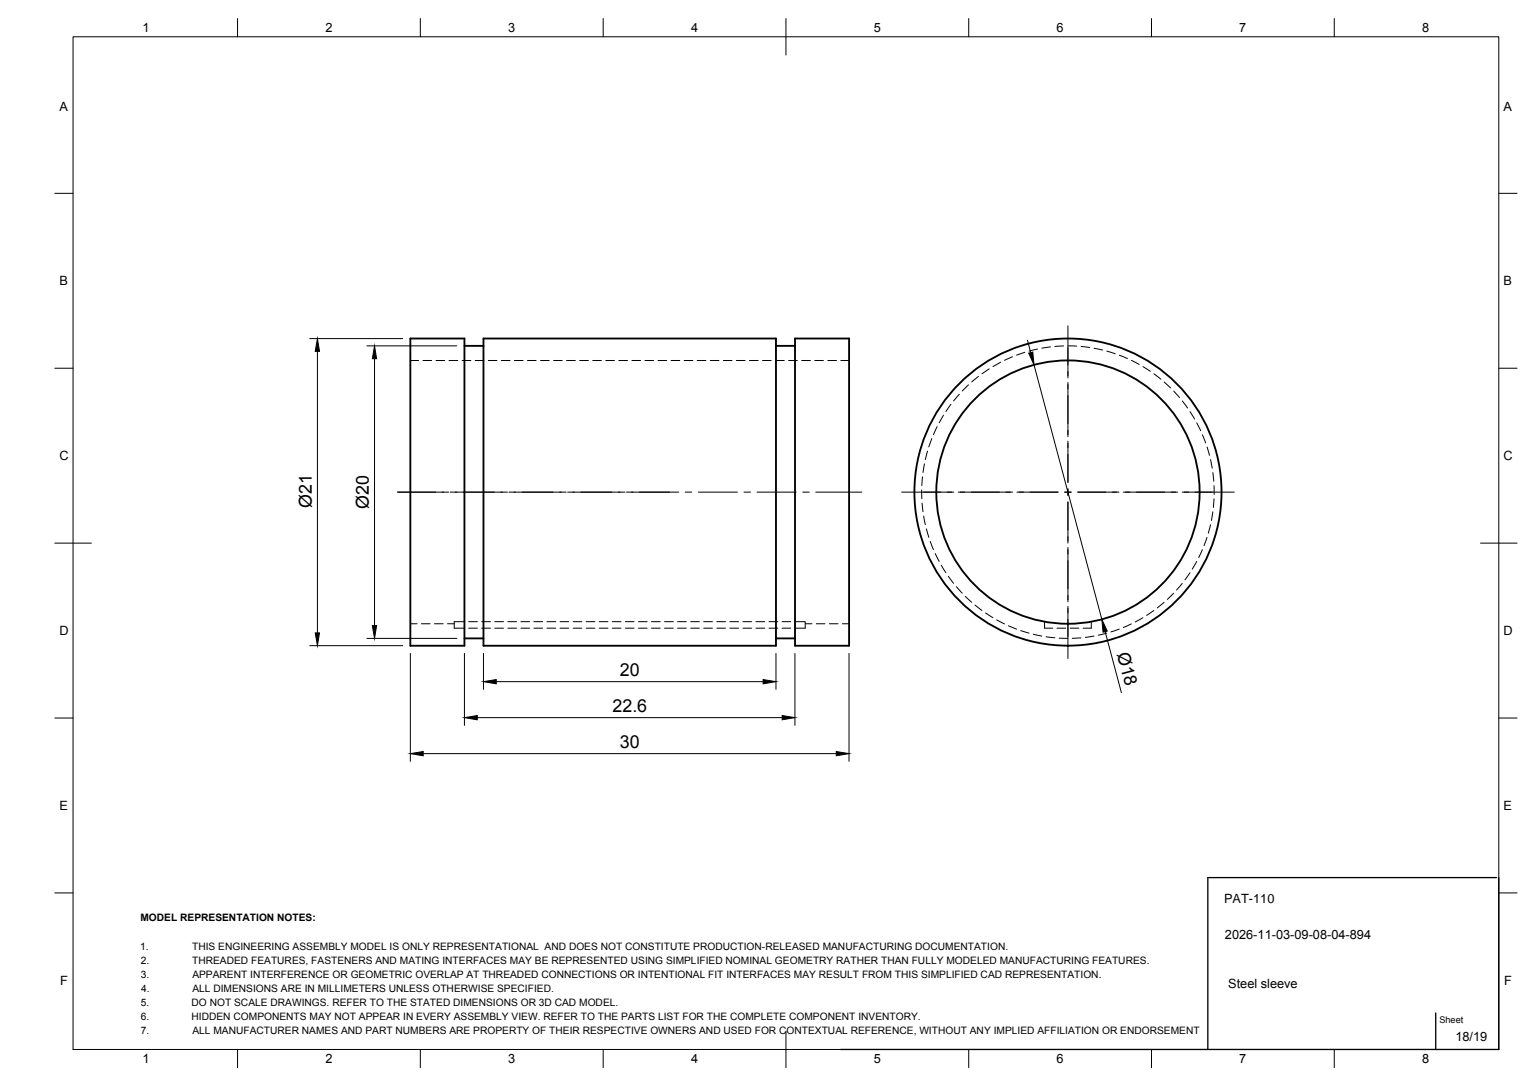
ISO-10303-21;
HEADER;
/* Generated by software containing ST-Developer
 * from STEP Tools, Inc. (www.steptools.com) 
 */

FILE_DESCRIPTION(
/* description */ ('Twin-shaft manual slide'),
/* implementation_level */ '2;1');

FILE_NAME(
/* name */ 'Steel sleeve.step',
/* time_stamp */ '2026-10-27T18:38:08-07:00',
/* author */ (''),
/* organization */ (''),
/* preprocessor_version */ 'ST-DEVELOPER v20.2',
/* originating_system */ 'Autodesk Translation Framework v15.17.0.0',
/* authorisation */ '');

FILE_SCHEMA (('AUTOMOTIVE_DESIGN { 1 0 10303 214 3 1 1 }'));
ENDSEC;

DATA;
#10=MECHANICAL_DESIGN_GEOMETRIC_PRESENTATION_REPRESENTATION('',(#284),#6463);
#252=SHAPE_REPRESENTATION_RELATIONSHIP('SRR','None',#6572,#268);
#268=ADVANCED_BREP_SHAPE_REPRESENTATION('',(#299),#6455);
#284=STYLED_ITEM('',(#6754),#299);
#299=MANIFOLD_SOLID_BREP('Body1',#3647);
#371=FACE_BOUND('',#917,.T.);
#372=FACE_BOUND('',#920,.T.);
#373=FACE_BOUND('',#923,.T.);
#374=FACE_BOUND('',#926,.T.);
#375=FACE_BOUND('',#929,.T.);
#376=FACE_BOUND('',#932,.T.);
#377=FACE_BOUND('',#934,.T.);
#466=PLANE('',#4046);
#467=PLANE('',#4048);
#468=PLANE('',#4049);
#469=PLANE('',#4051);
#470=PLANE('',#4052);
#471=PLANE('',#4053);
#472=PLANE('',#4058);
#473=PLANE('',#4062);
#474=PLANE('',#4066);
#475=PLANE('',#4070);
#476=PLANE('',#4074);
#637=FACE_OUTER_BOUND('',#911,.T.);
#638=FACE_OUTER_BOUND('',#912,.T.);
#639=FACE_OUTER_BOUND('',#913,.T.);
#640=FACE_OUTER_BOUND('',#914,.T.);
#641=FACE_OUTER_BOUND('',#915,.T.);
#642=FACE_OUTER_BOUND('',#916,.T.);
#643=FACE_OUTER_BOUND('',#918,.T.);
#644=FACE_OUTER_BOUND('',#919,.T.);
#645=FACE_OUTER_BOUND('',#921,.T.);
#646=FACE_OUTER_BOUND('',#922,.T.);
#647=FACE_OUTER_BOUND('',#924,.T.);
#648=FACE_OUTER_BOUND('',#925,.T.);
#649=FACE_OUTER_BOUND('',#927,.T.);
#650=FACE_OUTER_BOUND('',#928,.T.);
#651=FACE_OUTER_BOUND('',#930,.T.);
#652=FACE_OUTER_BOUND('',#931,.T.);
#653=FACE_OUTER_BOUND('',#933,.T.);
#911=EDGE_LOOP('',(#2994,#2995,#2996,#2997));
#912=EDGE_LOOP('',(#2998,#2999,#3000,#3001));
#913=EDGE_LOOP('',(#3002,#3003,#3004,#3005));
#914=EDGE_LOOP('',(#3006,#3007,#3008,#3009));
#915=EDGE_LOOP('',(#3010,#3011,#3012,#3013));
#916=EDGE_LOOP('',(#3014));
#917=EDGE_LOOP('',(#3015));
#918=EDGE_LOOP('',(#3016,#3017,#3018,#3019));
#919=EDGE_LOOP('',(#3020));
#920=EDGE_LOOP('',(#3021));
#921=EDGE_LOOP('',(#3022,#3023,#3024,#3025));
#922=EDGE_LOOP('',(#3026));
#923=EDGE_LOOP('',(#3027));
#924=EDGE_LOOP('',(#3028,#3029,#3030,#3031));
#925=EDGE_LOOP('',(#3032));
#926=EDGE_LOOP('',(#3033));
#927=EDGE_LOOP('',(#3034,#3035,#3036,#3037));
#928=EDGE_LOOP('',(#3038));
#929=EDGE_LOOP('',(#3039));
#930=EDGE_LOOP('',(#3040,#3041,#3042,#3043));
#931=EDGE_LOOP('',(#3044));
#932=EDGE_LOOP('',(#3045));
#933=EDGE_LOOP('',(#3046,#3047,#3048,#3049));
#934=EDGE_LOOP('',(#3050,#3051,#3052,#3053));
#1203=LINE('',#5966,#1489);
#1204=LINE('',#5968,#1490);
#1205=LINE('',#5969,#1491);
#1206=LINE('',#5972,#1492);
#1207=LINE('',#5974,#1493);
#1208=LINE('',#5975,#1494);
#1209=LINE('',#5980,#1495);
#1210=LINE('',#5981,#1496);
#1211=LINE('',#5983,#1497);
#1212=LINE('',#5984,#1498);
#1213=LINE('',#5994,#1499);
#1214=LINE('',#6001,#1500);
#1215=LINE('',#6008,#1501);
#1216=LINE('',#6015,#1502);
#1217=LINE('',#6022,#1503);
#1218=LINE('',#6027,#1504);
#1489=VECTOR('',#4859,1.);
#1490=VECTOR('',#4860,1.);
#1491=VECTOR('',#4861,1.);
#1492=VECTOR('',#4864,1.);
#1493=VECTOR('',#4865,1.);
#1494=VECTOR('',#4866,1.);
#1495=VECTOR('',#4871,1.);
#1496=VECTOR('',#4872,1.);
#1497=VECTOR('',#4875,1.);
#1498=VECTOR('',#4876,1.);
#1499=VECTOR('',#4889,1.05);
#1500=VECTOR('',#4898,1.);
#1501=VECTOR('',#4907,1.05);
#1502=VECTOR('',#4916,1.);
#1503=VECTOR('',#4925,1.05);
#1504=VECTOR('',#4932,0.9);
#1696=CIRCLE('',#4047,0.9);
#1697=CIRCLE('',#4050,0.9);
#1698=CIRCLE('',#4054,1.05);
#1699=CIRCLE('',#4055,0.9);
#1700=CIRCLE('',#4057,1.05);
#1701=CIRCLE('',#4059,1.);
#1702=CIRCLE('',#4061,1.);
#1703=CIRCLE('',#4063,1.05);
#1704=CIRCLE('',#4065,1.05);
#1705=CIRCLE('',#4067,1.);
#1706=CIRCLE('',#4069,1.);
#1707=CIRCLE('',#4071,1.05);
#1708=CIRCLE('',#4073,1.05);
#1709=CIRCLE('',#4075,0.9);
#1929=VERTEX_POINT('',#5962);
#1930=VERTEX_POINT('',#5963);
#1931=VERTEX_POINT('',#5965);
#1932=VERTEX_POINT('',#5967);
#1933=VERTEX_POINT('',#5971);
#1934=VERTEX_POINT('',#5973);
#1935=VERTEX_POINT('',#5977);
#1936=VERTEX_POINT('',#5979);
#1937=VERTEX_POINT('',#5987);
#1938=VERTEX_POINT('',#5989);
#1939=VERTEX_POINT('',#5992);
#1940=VERTEX_POINT('',#5996);
#1941=VERTEX_POINT('',#5999);
#1942=VERTEX_POINT('',#6003);
#1943=VERTEX_POINT('',#6006);
#1944=VERTEX_POINT('',#6010);
#1945=VERTEX_POINT('',#6013);
#1946=VERTEX_POINT('',#6017);
#1947=VERTEX_POINT('',#6020);
#1948=VERTEX_POINT('',#6024);
#2302=EDGE_CURVE('',#1929,#1930,#1696,.T.);
#2303=EDGE_CURVE('',#1931,#1929,#1203,.T.);
#2304=EDGE_CURVE('',#1932,#1931,#1204,.T.);
#2305=EDGE_CURVE('',#1930,#1932,#1205,.T.);
#2306=EDGE_CURVE('',#1930,#1933,#1206,.T.);
#2307=EDGE_CURVE('',#1934,#1932,#1207,.T.);
#2308=EDGE_CURVE('',#1934,#1933,#1208,.T.);
#2309=EDGE_CURVE('',#1933,#1935,#1697,.T.);
#2310=EDGE_CURVE('',#1936,#1934,#1209,.T.);
#2311=EDGE_CURVE('',#1935,#1936,#1210,.T.);
#2312=EDGE_CURVE('',#1935,#1929,#1211,.T.);
#2313=EDGE_CURVE('',#1936,#1931,#1212,.T.);
#2314=EDGE_CURVE('',#1937,#1937,#1698,.T.);
#2315=EDGE_CURVE('',#1938,#1938,#1699,.T.);
#2316=EDGE_CURVE('',#1939,#1939,#1700,.T.);
#2317=EDGE_CURVE('',#1939,#1937,#1213,.T.);
#2318=EDGE_CURVE('',#1940,#1940,#1701,.T.);
#2319=EDGE_CURVE('',#1941,#1941,#1702,.T.);
#2320=EDGE_CURVE('',#1941,#1940,#1214,.T.);
#2321=EDGE_CURVE('',#1942,#1942,#1703,.T.);
#2322=EDGE_CURVE('',#1943,#1943,#1704,.T.);
#2323=EDGE_CURVE('',#1943,#1942,#1215,.T.);
#2324=EDGE_CURVE('',#1944,#1944,#1705,.T.);
#2325=EDGE_CURVE('',#1945,#1945,#1706,.T.);
#2326=EDGE_CURVE('',#1945,#1944,#1216,.T.);
#2327=EDGE_CURVE('',#1946,#1946,#1707,.T.);
#2328=EDGE_CURVE('',#1947,#1947,#1708,.T.);
#2329=EDGE_CURVE('',#1947,#1946,#1217,.T.);
#2330=EDGE_CURVE('',#1948,#1948,#1709,.T.);
#2331=EDGE_CURVE('',#1948,#1938,#1218,.T.);
#2994=ORIENTED_EDGE('',*,*,#2302,.F.);
#2995=ORIENTED_EDGE('',*,*,#2303,.F.);
#2996=ORIENTED_EDGE('',*,*,#2304,.F.);
#2997=ORIENTED_EDGE('',*,*,#2305,.F.);
#2998=ORIENTED_EDGE('',*,*,#2306,.F.);
#2999=ORIENTED_EDGE('',*,*,#2305,.T.);
#3000=ORIENTED_EDGE('',*,*,#2307,.F.);
#3001=ORIENTED_EDGE('',*,*,#2308,.T.);
#3002=ORIENTED_EDGE('',*,*,#2309,.F.);
#3003=ORIENTED_EDGE('',*,*,#2308,.F.);
#3004=ORIENTED_EDGE('',*,*,#2310,.F.);
#3005=ORIENTED_EDGE('',*,*,#2311,.F.);
#3006=ORIENTED_EDGE('',*,*,#2312,.F.);
#3007=ORIENTED_EDGE('',*,*,#2311,.T.);
#3008=ORIENTED_EDGE('',*,*,#2313,.T.);
#3009=ORIENTED_EDGE('',*,*,#2303,.T.);
#3010=ORIENTED_EDGE('',*,*,#2313,.F.);
#3011=ORIENTED_EDGE('',*,*,#2310,.T.);
#3012=ORIENTED_EDGE('',*,*,#2307,.T.);
#3013=ORIENTED_EDGE('',*,*,#2304,.T.);
#3014=ORIENTED_EDGE('',*,*,#2314,.F.);
#3015=ORIENTED_EDGE('',*,*,#2315,.T.);
#3016=ORIENTED_EDGE('',*,*,#2316,.F.);
#3017=ORIENTED_EDGE('',*,*,#2317,.T.);
#3018=ORIENTED_EDGE('',*,*,#2314,.T.);
#3019=ORIENTED_EDGE('',*,*,#2317,.F.);
#3020=ORIENTED_EDGE('',*,*,#2316,.T.);
#3021=ORIENTED_EDGE('',*,*,#2318,.F.);
#3022=ORIENTED_EDGE('',*,*,#2319,.F.);
#3023=ORIENTED_EDGE('',*,*,#2320,.T.);
#3024=ORIENTED_EDGE('',*,*,#2318,.T.);
#3025=ORIENTED_EDGE('',*,*,#2320,.F.);
#3026=ORIENTED_EDGE('',*,*,#2321,.F.);
#3027=ORIENTED_EDGE('',*,*,#2319,.T.);
#3028=ORIENTED_EDGE('',*,*,#2322,.F.);
#3029=ORIENTED_EDGE('',*,*,#2323,.T.);
#3030=ORIENTED_EDGE('',*,*,#2321,.T.);
#3031=ORIENTED_EDGE('',*,*,#2323,.F.);
#3032=ORIENTED_EDGE('',*,*,#2322,.T.);
#3033=ORIENTED_EDGE('',*,*,#2324,.F.);
#3034=ORIENTED_EDGE('',*,*,#2325,.F.);
#3035=ORIENTED_EDGE('',*,*,#2326,.T.);
#3036=ORIENTED_EDGE('',*,*,#2324,.T.);
#3037=ORIENTED_EDGE('',*,*,#2326,.F.);
#3038=ORIENTED_EDGE('',*,*,#2327,.F.);
#3039=ORIENTED_EDGE('',*,*,#2325,.T.);
#3040=ORIENTED_EDGE('',*,*,#2328,.F.);
#3041=ORIENTED_EDGE('',*,*,#2329,.T.);
#3042=ORIENTED_EDGE('',*,*,#2327,.T.);
#3043=ORIENTED_EDGE('',*,*,#2329,.F.);
#3044=ORIENTED_EDGE('',*,*,#2328,.T.);
#3045=ORIENTED_EDGE('',*,*,#2330,.F.);
#3046=ORIENTED_EDGE('',*,*,#2330,.T.);
#3047=ORIENTED_EDGE('',*,*,#2331,.T.);
#3048=ORIENTED_EDGE('',*,*,#2315,.F.);
#3049=ORIENTED_EDGE('',*,*,#2331,.F.);
#3050=ORIENTED_EDGE('',*,*,#2309,.T.);
#3051=ORIENTED_EDGE('',*,*,#2312,.T.);
#3052=ORIENTED_EDGE('',*,*,#2302,.T.);
#3053=ORIENTED_EDGE('',*,*,#2306,.T.);
#3407=CYLINDRICAL_SURFACE('',#4056,1.05);
#3408=CYLINDRICAL_SURFACE('',#4060,1.);
#3409=CYLINDRICAL_SURFACE('',#4064,1.05);
#3410=CYLINDRICAL_SURFACE('',#4068,1.);
#3411=CYLINDRICAL_SURFACE('',#4072,1.05);
#3412=CYLINDRICAL_SURFACE('',#4076,0.9);
#3542=ADVANCED_FACE('',(#637),#466,.F.);
#3543=ADVANCED_FACE('',(#638),#467,.F.);
#3544=ADVANCED_FACE('',(#639),#468,.F.);
#3545=ADVANCED_FACE('',(#640),#469,.F.);
#3546=ADVANCED_FACE('',(#641),#470,.F.);
#3547=ADVANCED_FACE('',(#642,#371),#471,.T.);
#3548=ADVANCED_FACE('',(#643),#3407,.T.);
#3549=ADVANCED_FACE('',(#644,#372),#472,.T.);
#3550=ADVANCED_FACE('',(#645),#3408,.T.);
#3551=ADVANCED_FACE('',(#646,#373),#473,.T.);
#3552=ADVANCED_FACE('',(#647),#3409,.T.);
#3553=ADVANCED_FACE('',(#648,#374),#474,.T.);
#3554=ADVANCED_FACE('',(#649),#3410,.T.);
#3555=ADVANCED_FACE('',(#650,#375),#475,.T.);
#3556=ADVANCED_FACE('',(#651),#3411,.T.);
#3557=ADVANCED_FACE('',(#652,#376),#476,.T.);
#3558=ADVANCED_FACE('',(#653,#377),#3412,.F.);
#3647=CLOSED_SHELL('',(#3542,#3543,#3544,#3545,#3546,#3547,#3548,#3549,
#3550,#3551,#3552,#3553,#3554,#3555,#3556,#3557,#3558));
#4045=AXIS2_PLACEMENT_3D('',#5960,#4853,#4854);
#4046=AXIS2_PLACEMENT_3D('',#5961,#4855,#4856);
#4047=AXIS2_PLACEMENT_3D('',#5964,#4857,#4858);
#4048=AXIS2_PLACEMENT_3D('',#5970,#4862,#4863);
#4049=AXIS2_PLACEMENT_3D('',#5976,#4867,#4868);
#4050=AXIS2_PLACEMENT_3D('',#5978,#4869,#4870);
#4051=AXIS2_PLACEMENT_3D('',#5982,#4873,#4874);
#4052=AXIS2_PLACEMENT_3D('',#5985,#4877,#4878);
#4053=AXIS2_PLACEMENT_3D('',#5986,#4879,#4880);
#4054=AXIS2_PLACEMENT_3D('',#5988,#4881,#4882);
#4055=AXIS2_PLACEMENT_3D('',#5990,#4883,#4884);
#4056=AXIS2_PLACEMENT_3D('',#5991,#4885,#4886);
#4057=AXIS2_PLACEMENT_3D('',#5993,#4887,#4888);
#4058=AXIS2_PLACEMENT_3D('',#5995,#4890,#4891);
#4059=AXIS2_PLACEMENT_3D('',#5997,#4892,#4893);
#4060=AXIS2_PLACEMENT_3D('',#5998,#4894,#4895);
#4061=AXIS2_PLACEMENT_3D('',#6000,#4896,#4897);
#4062=AXIS2_PLACEMENT_3D('',#6002,#4899,#4900);
#4063=AXIS2_PLACEMENT_3D('',#6004,#4901,#4902);
#4064=AXIS2_PLACEMENT_3D('',#6005,#4903,#4904);
#4065=AXIS2_PLACEMENT_3D('',#6007,#4905,#4906);
#4066=AXIS2_PLACEMENT_3D('',#6009,#4908,#4909);
#4067=AXIS2_PLACEMENT_3D('',#6011,#4910,#4911);
#4068=AXIS2_PLACEMENT_3D('',#6012,#4912,#4913);
#4069=AXIS2_PLACEMENT_3D('',#6014,#4914,#4915);
#4070=AXIS2_PLACEMENT_3D('',#6016,#4917,#4918);
#4071=AXIS2_PLACEMENT_3D('',#6018,#4919,#4920);
#4072=AXIS2_PLACEMENT_3D('',#6019,#4921,#4922);
#4073=AXIS2_PLACEMENT_3D('',#6021,#4923,#4924);
#4074=AXIS2_PLACEMENT_3D('',#6023,#4926,#4927);
#4075=AXIS2_PLACEMENT_3D('',#6025,#4928,#4929);
#4076=AXIS2_PLACEMENT_3D('',#6026,#4930,#4931);
#4853=DIRECTION('axis',(0.,0.,1.));
#4854=DIRECTION('refdir',(1.,0.,0.));
#4855=DIRECTION('center_axis',(0.,1.,0.));
#4856=DIRECTION('ref_axis',(0.,0.,1.));
#4857=DIRECTION('center_axis',(0.,-1.,0.));
#4858=DIRECTION('ref_axis',(1.,0.,0.));
#4859=DIRECTION('',(-1.,0.,0.));
#4860=DIRECTION('',(0.,0.,-1.));
#4861=DIRECTION('',(1.,0.,0.));
#4862=DIRECTION('center_axis',(0.,0.,1.));
#4863=DIRECTION('ref_axis',(1.,0.,0.));
#4864=DIRECTION('',(0.,-1.,0.));
#4865=DIRECTION('',(0.,1.,0.));
#4866=DIRECTION('',(-1.,0.,0.));
#4867=DIRECTION('center_axis',(0.,-1.,0.));
#4868=DIRECTION('ref_axis',(0.,0.,-1.));
#4869=DIRECTION('center_axis',(0.,1.,0.));
#4870=DIRECTION('ref_axis',(1.,0.,0.));
#4871=DIRECTION('',(0.,0.,1.));
#4872=DIRECTION('',(1.,0.,0.));
#4873=DIRECTION('center_axis',(0.,0.,-1.));
#4874=DIRECTION('ref_axis',(-1.,0.,0.));
#4875=DIRECTION('',(0.,1.,0.));
#4876=DIRECTION('',(0.,1.,0.));
#4877=DIRECTION('center_axis',(1.,0.,0.));
#4878=DIRECTION('ref_axis',(0.,0.,-1.));
#4879=DIRECTION('center_axis',(0.,1.,0.));
#4880=DIRECTION('ref_axis',(0.,0.,1.));
#4881=DIRECTION('center_axis',(0.,-1.,0.));
#4882=DIRECTION('ref_axis',(1.,0.,0.));
#4883=DIRECTION('center_axis',(0.,-1.,0.));
#4884=DIRECTION('ref_axis',(1.,0.,0.));
#4885=DIRECTION('center_axis',(0.,-1.,0.));
#4886=DIRECTION('ref_axis',(1.,0.,0.));
#4887=DIRECTION('center_axis',(0.,-1.,0.));
#4888=DIRECTION('ref_axis',(1.,0.,0.));
#4889=DIRECTION('',(0.,1.,0.));
#4890=DIRECTION('center_axis',(0.,-1.,0.));
#4891=DIRECTION('ref_axis',(0.,0.,-1.));
#4892=DIRECTION('center_axis',(0.,-1.,0.));
#4893=DIRECTION('ref_axis',(1.,0.,0.));
#4894=DIRECTION('center_axis',(0.,-1.,0.));
#4895=DIRECTION('ref_axis',(1.,0.,0.));
#4896=DIRECTION('center_axis',(0.,-1.,0.));
#4897=DIRECTION('ref_axis',(1.,0.,0.));
#4898=DIRECTION('',(0.,1.,0.));
#4899=DIRECTION('center_axis',(0.,1.,0.));
#4900=DIRECTION('ref_axis',(0.,0.,1.));
#4901=DIRECTION('center_axis',(0.,-1.,0.));
#4902=DIRECTION('ref_axis',(1.,0.,0.));
#4903=DIRECTION('center_axis',(0.,-1.,0.));
#4904=DIRECTION('ref_axis',(1.,0.,0.));
#4905=DIRECTION('center_axis',(0.,-1.,0.));
#4906=DIRECTION('ref_axis',(1.,0.,0.));
#4907=DIRECTION('',(0.,1.,0.));
#4908=DIRECTION('center_axis',(0.,-1.,0.));
#4909=DIRECTION('ref_axis',(0.,0.,-1.));
#4910=DIRECTION('center_axis',(0.,-1.,0.));
#4911=DIRECTION('ref_axis',(1.,0.,0.));
#4912=DIRECTION('center_axis',(0.,-1.,0.));
#4913=DIRECTION('ref_axis',(1.,0.,0.));
#4914=DIRECTION('center_axis',(0.,-1.,0.));
#4915=DIRECTION('ref_axis',(1.,0.,0.));
#4916=DIRECTION('',(0.,1.,0.));
#4917=DIRECTION('center_axis',(0.,1.,0.));
#4918=DIRECTION('ref_axis',(0.,0.,1.));
#4919=DIRECTION('center_axis',(0.,-1.,0.));
#4920=DIRECTION('ref_axis',(1.,0.,0.));
#4921=DIRECTION('center_axis',(0.,-1.,0.));
#4922=DIRECTION('ref_axis',(1.,0.,0.));
#4923=DIRECTION('center_axis',(0.,-1.,0.));
#4924=DIRECTION('ref_axis',(1.,0.,0.));
#4925=DIRECTION('',(0.,1.,0.));
#4926=DIRECTION('center_axis',(0.,-1.,0.));
#4927=DIRECTION('ref_axis',(0.,0.,-1.));
#4928=DIRECTION('center_axis',(0.,-1.,0.));
#4929=DIRECTION('ref_axis',(1.,0.,0.));
#4930=DIRECTION('center_axis',(0.,-1.,0.));
#4931=DIRECTION('ref_axis',(1.,0.,0.));
#4932=DIRECTION('',(0.,1.,0.));
#5960=CARTESIAN_POINT('',(0.,0.,0.));
#5961=CARTESIAN_POINT('Origin',(0.75,1.2,0.));
#5962=CARTESIAN_POINT('',(0.885663593019381,1.2,-0.16));
#5963=CARTESIAN_POINT('',(0.885663593019381,1.2,0.16));
#5964=CARTESIAN_POINT('Origin',(0.,1.2,0.));
#5965=CARTESIAN_POINT('',(0.93,1.2,-0.16));
#5966=CARTESIAN_POINT('',(0.93,1.2,-0.16));
#5967=CARTESIAN_POINT('',(0.93,1.2,0.16));
#5968=CARTESIAN_POINT('',(0.93,1.2,0.16));
#5969=CARTESIAN_POINT('',(0.57,1.2,0.16));
#5970=CARTESIAN_POINT('Origin',(0.57,0.,0.16));
#5971=CARTESIAN_POINT('',(0.885663593019381,-1.2,0.16));
#5972=CARTESIAN_POINT('',(0.885663593019381,0.,0.16));
#5973=CARTESIAN_POINT('',(0.93,-1.2,0.16));
#5974=CARTESIAN_POINT('',(0.93,0.,0.16));
#5975=CARTESIAN_POINT('',(0.57,-1.2,0.16));
#5976=CARTESIAN_POINT('Origin',(0.75,-1.2,0.));
#5977=CARTESIAN_POINT('',(0.885663593019381,-1.2,-0.16));
#5978=CARTESIAN_POINT('Origin',(0.,-1.2,0.));
#5979=CARTESIAN_POINT('',(0.93,-1.2,-0.16));
#5980=CARTESIAN_POINT('',(0.93,-1.2,0.16));
#5981=CARTESIAN_POINT('',(0.93,-1.2,-0.16));
#5982=CARTESIAN_POINT('Origin',(0.93,0.,-0.16));
#5983=CARTESIAN_POINT('',(0.885663593019381,0.,-0.16));
#5984=CARTESIAN_POINT('',(0.93,0.,-0.16));
#5985=CARTESIAN_POINT('Origin',(0.93,0.,0.16));
#5986=CARTESIAN_POINT('Origin',(1.05,1.5,0.));
#5987=CARTESIAN_POINT('',(-1.05,1.5,-1.28587913910472E-16));
#5988=CARTESIAN_POINT('Origin',(0.,1.5,0.));
#5989=CARTESIAN_POINT('',(-0.9,1.5,-1.10218211923262E-16));
#5990=CARTESIAN_POINT('Origin',(0.,1.5,0.));
#5991=CARTESIAN_POINT('Origin',(0.,1.315,0.));
#5992=CARTESIAN_POINT('',(-1.05,1.13,-1.28587913910472E-16));
#5993=CARTESIAN_POINT('Origin',(0.,1.13,0.));
#5994=CARTESIAN_POINT('',(-1.05,1.315,-1.28587913910472E-16));
#5995=CARTESIAN_POINT('Origin',(1.,1.13,0.));
#5996=CARTESIAN_POINT('',(-1.,1.13,-1.22464679914735E-16));
#5997=CARTESIAN_POINT('Origin',(0.,1.13,0.));
#5998=CARTESIAN_POINT('Origin',(0.,1.065,0.));
#5999=CARTESIAN_POINT('',(-1.,1.,-1.22464679914735E-16));
#6000=CARTESIAN_POINT('Origin',(0.,1.,0.));
#6001=CARTESIAN_POINT('',(-1.,1.065,-1.22464679914735E-16));
#6002=CARTESIAN_POINT('Origin',(1.05,1.,0.));
#6003=CARTESIAN_POINT('',(-1.05,1.,-1.28587913910472E-16));
#6004=CARTESIAN_POINT('Origin',(0.,1.,0.));
#6005=CARTESIAN_POINT('Origin',(0.,0.,0.));
#6006=CARTESIAN_POINT('',(-1.05,-1.,-1.28587913910472E-16));
#6007=CARTESIAN_POINT('Origin',(0.,-1.,0.));
#6008=CARTESIAN_POINT('',(-1.05,0.,-1.28587913910472E-16));
#6009=CARTESIAN_POINT('Origin',(1.,-1.,0.));
#6010=CARTESIAN_POINT('',(-1.,-1.,-1.22464679914735E-16));
#6011=CARTESIAN_POINT('Origin',(0.,-1.,0.));
#6012=CARTESIAN_POINT('Origin',(0.,-1.065,0.));
#6013=CARTESIAN_POINT('',(-1.,-1.13,-1.22464679914735E-16));
#6014=CARTESIAN_POINT('Origin',(0.,-1.13,0.));
#6015=CARTESIAN_POINT('',(-1.,-1.065,-1.22464679914735E-16));
#6016=CARTESIAN_POINT('Origin',(1.05,-1.13,0.));
#6017=CARTESIAN_POINT('',(-1.05,-1.13,-1.28587913910472E-16));
#6018=CARTESIAN_POINT('Origin',(0.,-1.13,0.));
#6019=CARTESIAN_POINT('Origin',(0.,-1.315,0.));
#6020=CARTESIAN_POINT('',(-1.05,-1.5,-1.28587913910472E-16));
#6021=CARTESIAN_POINT('Origin',(0.,-1.5,0.));
#6022=CARTESIAN_POINT('',(-1.05,-1.315,-1.28587913910472E-16));
#6023=CARTESIAN_POINT('Origin',(0.9,-1.5,0.));
#6024=CARTESIAN_POINT('',(-0.9,-1.5,-1.10218211923262E-16));
#6025=CARTESIAN_POINT('Origin',(0.,-1.5,0.));
#6026=CARTESIAN_POINT('Origin',(0.,0.,0.));
#6027=CARTESIAN_POINT('',(-0.9,0.,-1.10218211923262E-16));
#6434=UNCERTAINTY_MEASURE_WITH_UNIT(LENGTH_MEASURE(0.001),#6464,
'DISTANCE_ACCURACY_VALUE',
'Maximum model space distance between geometric entities at asserted c
onnectivities');
#6442=UNCERTAINTY_MEASURE_WITH_UNIT(LENGTH_MEASURE(0.001),#6464,
'DISTANCE_ACCURACY_VALUE',
'Maximum model space distance between geometric entities at asserted c
onnectivities');
#6455=(
GEOMETRIC_REPRESENTATION_CONTEXT(3)
GLOBAL_UNCERTAINTY_ASSIGNED_CONTEXT((#6434))
GLOBAL_UNIT_ASSIGNED_CONTEXT((#6464,#6466,#6467))
REPRESENTATION_CONTEXT('','3D')
);
#6463=(
GEOMETRIC_REPRESENTATION_CONTEXT(3)
GLOBAL_UNCERTAINTY_ASSIGNED_CONTEXT((#6442))
GLOBAL_UNIT_ASSIGNED_CONTEXT((#6464,#6466,#6467))
REPRESENTATION_CONTEXT('','3D')
);
#6464=(
LENGTH_UNIT()
NAMED_UNIT(*)
SI_UNIT(.CENTI.,.METRE.)
);
#6466=(
NAMED_UNIT(*)
PLANE_ANGLE_UNIT()
SI_UNIT($,.RADIAN.)
);
#6467=(
NAMED_UNIT(*)
SI_UNIT($,.STERADIAN.)
SOLID_ANGLE_UNIT()
);
#6480=SHAPE_DEFINITION_REPRESENTATION(#6500,#6572);
#6500=PRODUCT_DEFINITION_SHAPE('',$,#6593);
#6572=SHAPE_REPRESENTATION('',(#4045),#6455);
#6580=PRODUCT_DEFINITION_CONTEXT('part definition',#6642,'design');
#6593=PRODUCT_DEFINITION('Steel sleeve','Steel sleeve',#6613,#6580);
#6613=PRODUCT_DEFINITION_FORMATION('',$,#6656);
#6642=APPLICATION_CONTEXT(
'Core Data for Automotive Mechanical Design Process');
#6643=PRODUCT_CONTEXT('part definition',#6642,'mechanical');
#6656=PRODUCT('Steel sleeve','Steel sleeve','Steel sleeve',(#6643));
#6748=COLOUR_RGB('Off White',0.89,0.88,0.83);
#6749=FILL_AREA_STYLE_COLOUR('',#6748);
#6750=FILL_AREA_STYLE('',(#6749));
#6751=SURFACE_STYLE_FILL_AREA(#6750);
#6752=SURFACE_SIDE_STYLE('',(#6751));
#6753=SURFACE_STYLE_USAGE(.BOTH.,#6752);
#6754=PRESENTATION_STYLE_ASSIGNMENT((#6753));
ENDSEC;
END-ISO-10303-21;
